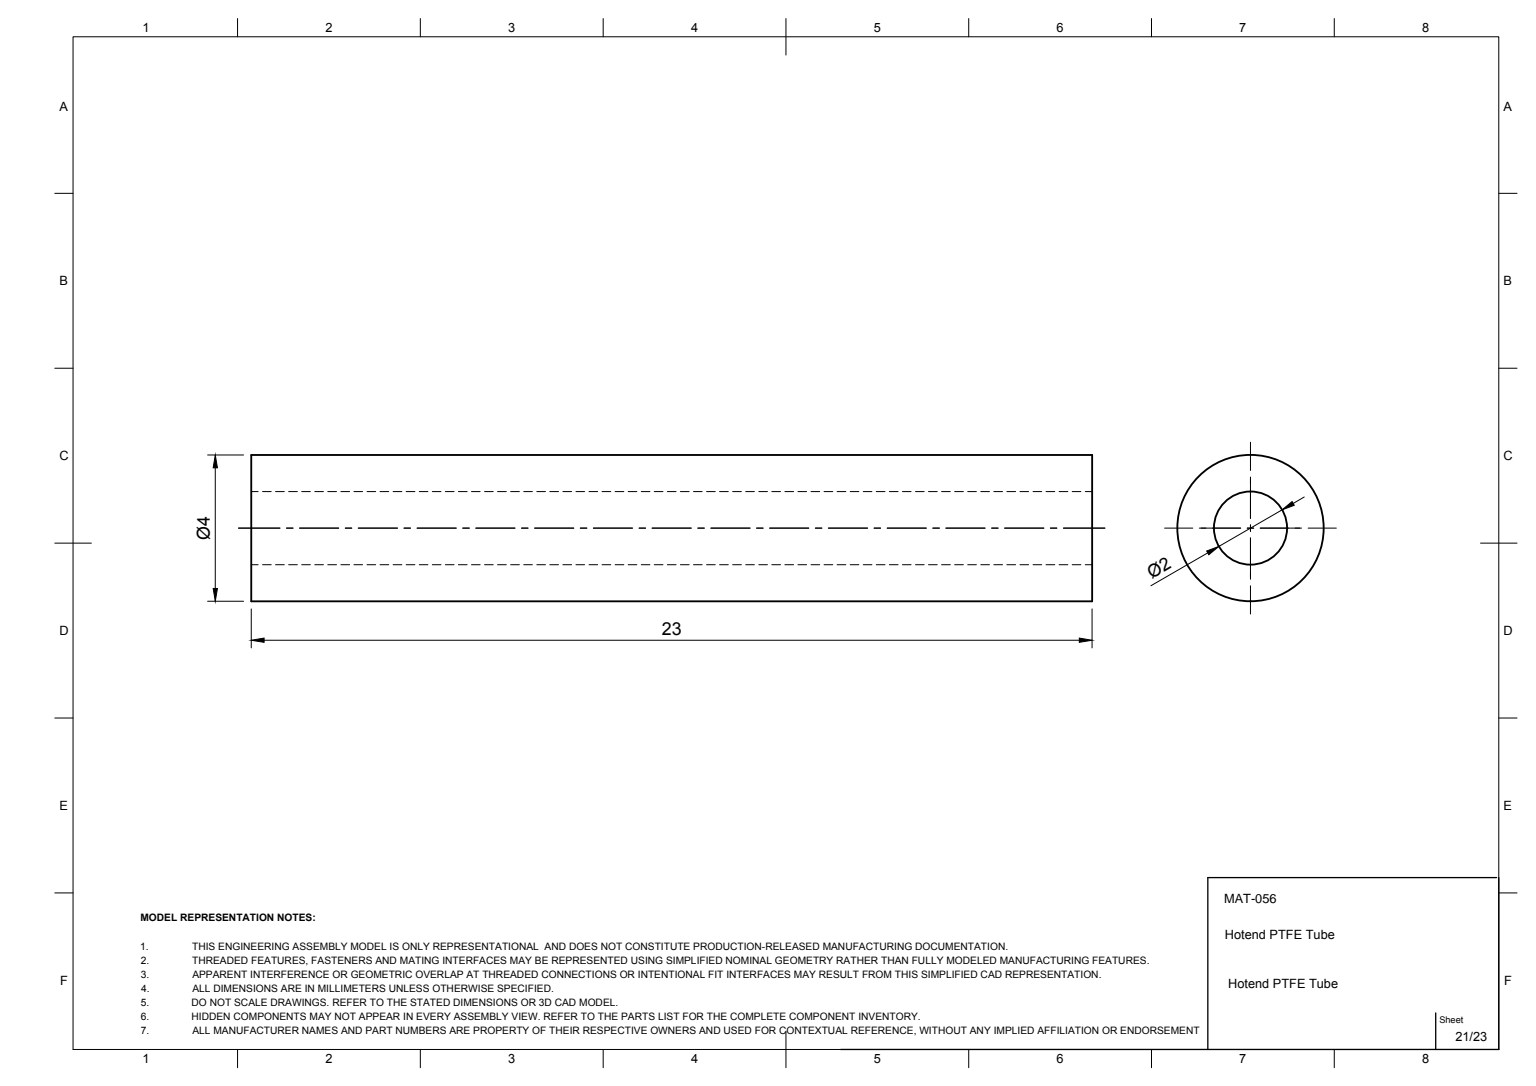
ISO-10303-21;
HEADER;
/* Generated by software containing ST-Developer
 * from STEP Tools, Inc. (www.steptools.com) 
 */

FILE_DESCRIPTION(
/* description */ (''),
/* implementation_level */ '2;1');

FILE_NAME(
/* name */ 'Hotend PTFE Tube.step',
/* time_stamp */ '2026-10-28T16:47:13+01:00',
/* author */ (''),
/* organization */ (''),
/* preprocessor_version */ 'ST-DEVELOPER v20.2',
/* originating_system */ 'Autodesk Translation Framework v15.17.0.0',
/* authorisation */ '');

FILE_SCHEMA (('AUTOMOTIVE_DESIGN { 1 0 10303 214 3 1 1 }'));
ENDSEC;

DATA;
#10=MECHANICAL_DESIGN_GEOMETRIC_PRESENTATION_REPRESENTATION('',(#4611),#459242);
#4423=SHAPE_REPRESENTATION_RELATIONSHIP('SRR','None',#459350,#4444);
#4444=ADVANCED_BREP_SHAPE_REPRESENTATION('',(#4491),#459239);
#4491=MANIFOLD_SOLID_BREP('Body1',#94669);
#4611=STYLED_ITEM('',(#459540),#4491);
#5264=FACE_BOUND('',#18040,.T.);
#5265=FACE_BOUND('',#18044,.T.);
#6134=PLANE('',#105432);
#6135=PLANE('',#105439);
#12080=FACE_OUTER_BOUND('',#18039,.T.);
#12081=FACE_OUTER_BOUND('',#18041,.T.);
#12082=FACE_OUTER_BOUND('',#18042,.T.);
#12083=FACE_OUTER_BOUND('',#18043,.T.);
#18039=EDGE_LOOP('',(#86696));
#18040=EDGE_LOOP('',(#86697));
#18041=EDGE_LOOP('',(#86698,#86699,#86700,#86701));
#18042=EDGE_LOOP('',(#86702,#86703,#86704,#86705));
#18043=EDGE_LOOP('',(#86706));
#18044=EDGE_LOOP('',(#86707));
#23463=CIRCLE('',#105433,2.);
#23464=CIRCLE('',#105434,1.);
#23465=CIRCLE('',#105436,1.);
#23466=CIRCLE('',#105438,2.);
#30740=LINE('',#457726,#34542);
#30741=LINE('',#457730,#34543);
#34542=VECTOR('',#130334,1.);
#34543=VECTOR('',#130339,2.);
#43407=VERTEX_POINT('',#457719);
#43408=VERTEX_POINT('',#457721);
#43409=VERTEX_POINT('',#457724);
#43410=VERTEX_POINT('',#457728);
#57850=EDGE_CURVE('',#43407,#43407,#23463,.T.);
#57851=EDGE_CURVE('',#43408,#43408,#23464,.T.);
#57852=EDGE_CURVE('',#43409,#43409,#23465,.T.);
#57853=EDGE_CURVE('',#43409,#43408,#30740,.T.);
#57854=EDGE_CURVE('',#43410,#43410,#23466,.T.);
#57855=EDGE_CURVE('',#43410,#43407,#30741,.T.);
#86696=ORIENTED_EDGE('',*,*,#57850,.T.);
#86697=ORIENTED_EDGE('',*,*,#57851,.T.);
#86698=ORIENTED_EDGE('',*,*,#57852,.F.);
#86699=ORIENTED_EDGE('',*,*,#57853,.T.);
#86700=ORIENTED_EDGE('',*,*,#57851,.F.);
#86701=ORIENTED_EDGE('',*,*,#57853,.F.);
#86702=ORIENTED_EDGE('',*,*,#57854,.F.);
#86703=ORIENTED_EDGE('',*,*,#57855,.T.);
#86704=ORIENTED_EDGE('',*,*,#57850,.F.);
#86705=ORIENTED_EDGE('',*,*,#57855,.F.);
#86706=ORIENTED_EDGE('',*,*,#57854,.T.);
#86707=ORIENTED_EDGE('',*,*,#57852,.T.);
#88789=CYLINDRICAL_SURFACE('',#105435,1.);
#88790=CYLINDRICAL_SURFACE('',#105437,2.);
#94544=ADVANCED_FACE('',(#12080,#5264),#6134,.F.);
#94545=ADVANCED_FACE('',(#12081),#88789,.F.);
#94546=ADVANCED_FACE('',(#12082),#88790,.T.);
#94547=ADVANCED_FACE('',(#12083,#5265),#6135,.T.);
#94669=CLOSED_SHELL('',(#94544,#94545,#94546,#94547));
#105431=AXIS2_PLACEMENT_3D('',#457717,#130322,#130323);
#105432=AXIS2_PLACEMENT_3D('',#457718,#130324,#130325);
#105433=AXIS2_PLACEMENT_3D('',#457720,#130326,#130327);
#105434=AXIS2_PLACEMENT_3D('',#457722,#130328,#130329);
#105435=AXIS2_PLACEMENT_3D('',#457723,#130330,#130331);
#105436=AXIS2_PLACEMENT_3D('',#457725,#130332,#130333);
#105437=AXIS2_PLACEMENT_3D('',#457727,#130335,#130336);
#105438=AXIS2_PLACEMENT_3D('',#457729,#130337,#130338);
#105439=AXIS2_PLACEMENT_3D('',#457731,#130340,#130341);
#130322=DIRECTION('axis',(0.,0.,1.));
#130323=DIRECTION('refdir',(1.,0.,0.));
#130324=DIRECTION('center_axis',(-1.07601673699754E-16,-5.16454430761843E-15,
-1.));
#130325=DIRECTION('ref_axis',(1.,1.29806344583732E-24,-1.07601673699754E-16));
#130326=DIRECTION('center_axis',(1.07601673699754E-16,5.16454430761843E-15,
1.));
#130327=DIRECTION('ref_axis',(1.,1.29806344583732E-24,-1.07601673699754E-16));
#130328=DIRECTION('center_axis',(-1.07601673699754E-16,-5.16454430761843E-15,
-1.));
#130329=DIRECTION('ref_axis',(1.,1.29806344583732E-24,-1.07601673699754E-16));
#130330=DIRECTION('center_axis',(-9.91270557701033E-17,-5.16454430759884E-15,
-1.));
#130331=DIRECTION('ref_axis',(1.,1.29806348960486E-24,-9.91270557701033E-17));
#130332=DIRECTION('center_axis',(1.07601673699754E-16,5.16454430761843E-15,
1.));
#130333=DIRECTION('ref_axis',(1.,1.29806344583732E-24,-1.07601673699754E-16));
#130334=DIRECTION('',(9.91270557701033E-17,5.16454430759884E-15,1.));
#130335=DIRECTION('center_axis',(-9.91270557701033E-17,-5.16454430759884E-15,
-1.));
#130336=DIRECTION('ref_axis',(1.,1.29806348960486E-24,-9.91270557701033E-17));
#130337=DIRECTION('center_axis',(-1.07601673699754E-16,-5.16454430761843E-15,
-1.));
#130338=DIRECTION('ref_axis',(1.,1.29806344583732E-24,-1.07601673699754E-16));
#130339=DIRECTION('',(9.91270557701033E-17,5.16454430759884E-15,1.));
#130340=DIRECTION('center_axis',(-1.07601673699754E-16,-5.16454430761843E-15,
-1.));
#130341=DIRECTION('ref_axis',(1.,1.29806344583732E-24,-1.07601673699754E-16));
#457717=CARTESIAN_POINT('',(0.,0.,0.));
#457718=CARTESIAN_POINT('Origin',(1.66533478931514E-15,-5.24520618636721E-7,
16.));
#457719=CARTESIAN_POINT('',(-2.,-5.24520618391792E-7,16.));
#457720=CARTESIAN_POINT('Origin',(1.66533478931514E-15,-5.24520618636721E-7,
16.));
#457721=CARTESIAN_POINT('',(-0.999999999999998,-5.24520618514257E-7,16.));
#457722=CARTESIAN_POINT('Origin',(1.66533478931514E-15,-5.24520618636721E-7,
16.));
#457723=CARTESIAN_POINT('Origin',(2.52377408738871E-22,-5.2452070126943E-7,
3.10862446895044E-14));
#457724=CARTESIAN_POINT('',(-1.,-5.24520737298776E-7,-6.99999999999997));
#457725=CARTESIAN_POINT('Origin',(-6.93889138013314E-16,-5.2452073742124E-7,
-6.99999999999997));
#457726=CARTESIAN_POINT('',(-1.,-5.24520701146966E-7,3.11853717452745E-14));
#457727=CARTESIAN_POINT('Origin',(2.52377408738871E-22,-5.2452070126943E-7,
3.10862446895044E-14));
#457728=CARTESIAN_POINT('',(-2.,-5.24520737176311E-7,-6.99999999999997));
#457729=CARTESIAN_POINT('Origin',(-6.93889138013314E-16,-5.2452073742124E-7,
-6.99999999999997));
#457730=CARTESIAN_POINT('',(-2.,-5.24520701024501E-7,3.12844988010446E-14));
#457731=CARTESIAN_POINT('Origin',(-6.93889138013314E-16,-5.2452073742124E-7,
-6.99999999999997));
#459213=UNCERTAINTY_MEASURE_WITH_UNIT(LENGTH_MEASURE(0.01),#459243,
'DISTANCE_ACCURACY_VALUE',
'Maximum model space distance between geometric entities at asserted c
onnectivities');
#459216=UNCERTAINTY_MEASURE_WITH_UNIT(LENGTH_MEASURE(0.01),#459243,
'DISTANCE_ACCURACY_VALUE',
'Maximum model space distance between geometric entities at asserted c
onnectivities');
#459239=(
GEOMETRIC_REPRESENTATION_CONTEXT(3)
GLOBAL_UNCERTAINTY_ASSIGNED_CONTEXT((#459213))
GLOBAL_UNIT_ASSIGNED_CONTEXT((#459243,#459245,#459246))
REPRESENTATION_CONTEXT('','3D')
);
#459242=(
GEOMETRIC_REPRESENTATION_CONTEXT(3)
GLOBAL_UNCERTAINTY_ASSIGNED_CONTEXT((#459216))
GLOBAL_UNIT_ASSIGNED_CONTEXT((#459243,#459245,#459246))
REPRESENTATION_CONTEXT('','3D')
);
#459243=(
LENGTH_UNIT()
NAMED_UNIT(*)
SI_UNIT(.MILLI.,.METRE.)
);
#459245=(
NAMED_UNIT(*)
PLANE_ANGLE_UNIT()
SI_UNIT($,.RADIAN.)
);
#459246=(
NAMED_UNIT(*)
SI_UNIT($,.STERADIAN.)
SOLID_ANGLE_UNIT()
);
#459269=SHAPE_DEFINITION_REPRESENTATION(#459296,#459350);
#459296=PRODUCT_DEFINITION_SHAPE('',$,#459376);
#459350=SHAPE_REPRESENTATION('',(#105431),#459239);
#459353=PRODUCT_DEFINITION_CONTEXT('part definition',#459430,'design');
#459376=PRODUCT_DEFINITION('Hotend PTFE Tube','Hotend PTFE Tube',#459401,
#459353);
#459401=PRODUCT_DEFINITION_FORMATION('',$,#459454);
#459430=APPLICATION_CONTEXT(
'Core Data for Automotive Mechanical Design Process');
#459431=PRODUCT_CONTEXT('part definition',#459430,'mechanical');
#459454=PRODUCT('Hotend PTFE Tube','Hotend PTFE Tube',$,(#459431));
#459534=COLOUR_RGB('Off White',0.89,0.88,0.83);
#459535=FILL_AREA_STYLE_COLOUR('',#459534);
#459536=FILL_AREA_STYLE('',(#459535));
#459537=SURFACE_STYLE_FILL_AREA(#459536);
#459538=SURFACE_SIDE_STYLE('',(#459537));
#459539=SURFACE_STYLE_USAGE(.BOTH.,#459538);
#459540=PRESENTATION_STYLE_ASSIGNMENT((#459539));
ENDSEC;
END-ISO-10303-21;
